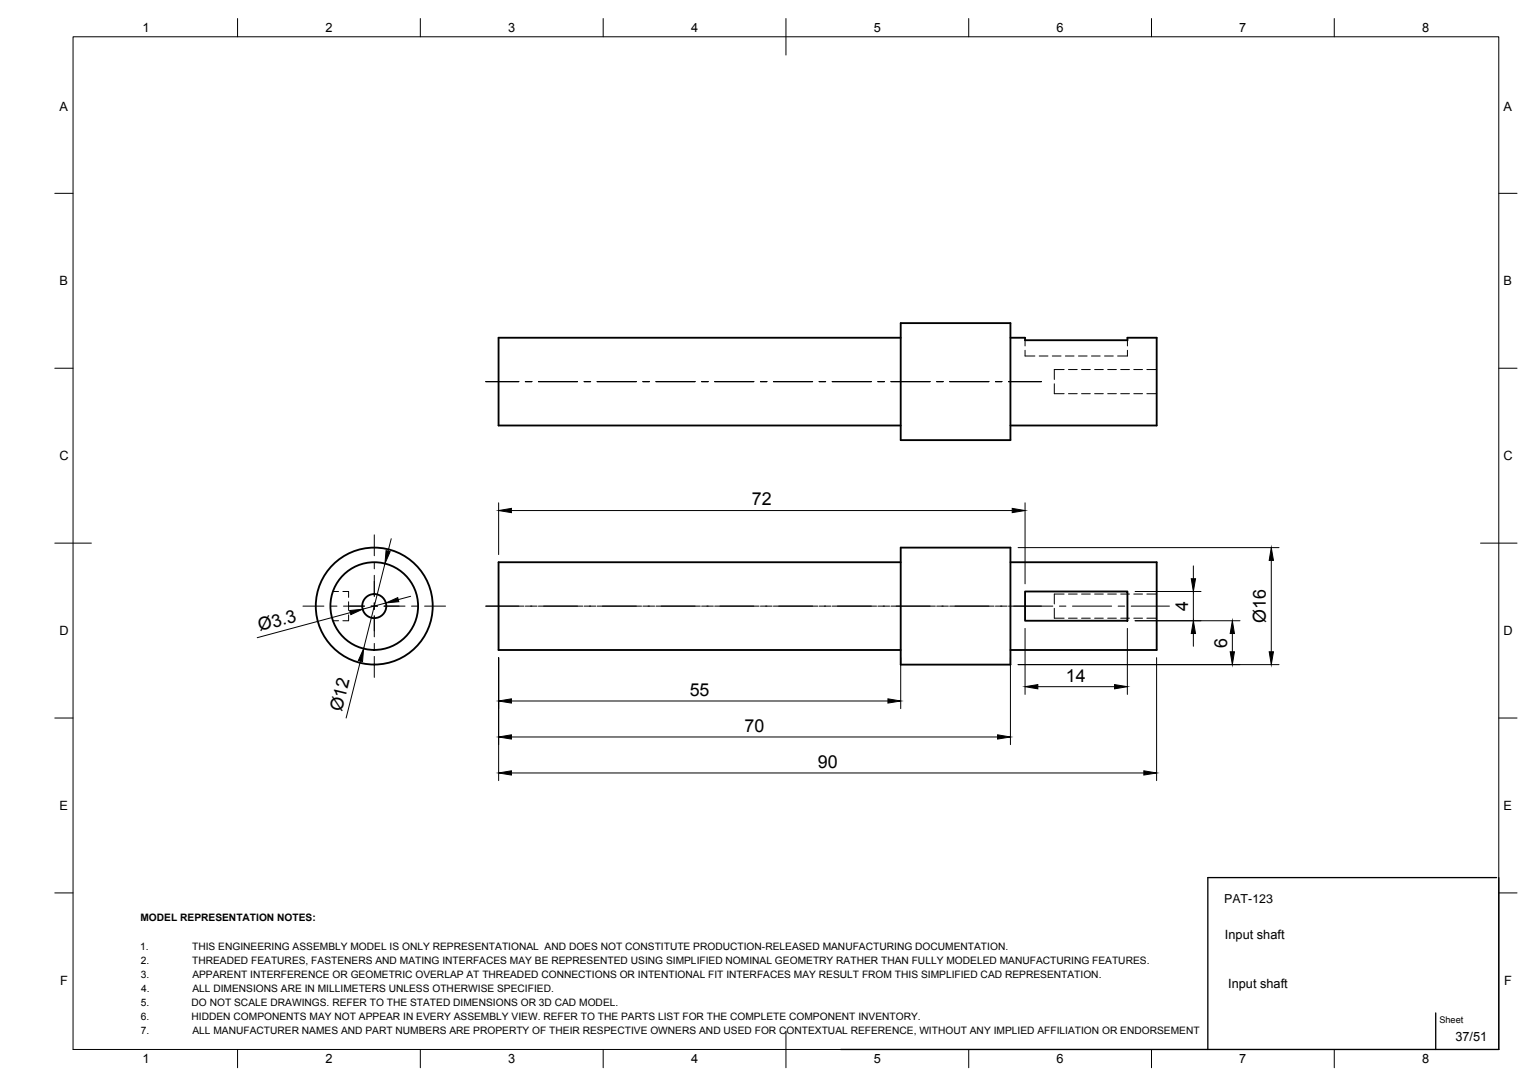
ISO-10303-21;
HEADER;
/* Generated by software containing ST-Developer
 * from STEP Tools, Inc. (www.steptools.com) 
 */

FILE_DESCRIPTION(
/* description */ ('Worm-less right-angle friction wheel drive'),
/* implementation_level */ '2;1');

FILE_NAME(
/* name */ 'Input shaft.step',
/* time_stamp */ '2026-10-28T03:22:36-07:00',
/* author */ (''),
/* organization */ (''),
/* preprocessor_version */ 'ST-DEVELOPER v20.2',
/* originating_system */ 'Autodesk Translation Framework v15.17.0.0',
/* authorisation */ '');

FILE_SCHEMA (('AUTOMOTIVE_DESIGN { 1 0 10303 214 3 1 1 }'));
ENDSEC;

DATA;
#10=MECHANICAL_DESIGN_GEOMETRIC_PRESENTATION_REPRESENTATION('',(#650),#17046);
#549=SHAPE_REPRESENTATION_RELATIONSHIP('SRR','None',#17294,#596);
#596=ADVANCED_BREP_SHAPE_REPRESENTATION('',(#701),#17030);
#650=STYLED_ITEM('',(#17591),#701);
#701=MANIFOLD_SOLID_BREP('Body1',#8208);
#919=FACE_BOUND('',#2229,.T.);
#920=FACE_BOUND('',#2231,.T.);
#921=FACE_BOUND('',#2235,.T.);
#922=FACE_BOUND('',#2237,.T.);
#1125=PLANE('',#9460);
#1126=PLANE('',#9461);
#1127=PLANE('',#9462);
#1128=PLANE('',#9464);
#1129=PLANE('',#9465);
#1130=PLANE('',#9466);
#1131=PLANE('',#9468);
#1132=PLANE('',#9471);
#1133=PLANE('',#9479);
#1134=PLANE('',#9480);
#1551=FACE_OUTER_BOUND('',#2221,.T.);
#1552=FACE_OUTER_BOUND('',#2222,.T.);
#1553=FACE_OUTER_BOUND('',#2223,.T.);
#1554=FACE_OUTER_BOUND('',#2224,.T.);
#1555=FACE_OUTER_BOUND('',#2225,.T.);
#1556=FACE_OUTER_BOUND('',#2226,.T.);
#1557=FACE_OUTER_BOUND('',#2227,.T.);
#1558=FACE_OUTER_BOUND('',#2228,.T.);
#1559=FACE_OUTER_BOUND('',#2230,.T.);
#1560=FACE_OUTER_BOUND('',#2232,.T.);
#1561=FACE_OUTER_BOUND('',#2233,.T.);
#1562=FACE_OUTER_BOUND('',#2234,.T.);
#1563=FACE_OUTER_BOUND('',#2236,.T.);
#1564=FACE_OUTER_BOUND('',#2238,.T.);
#2221=EDGE_LOOP('',(#7038,#7039,#7040,#7041));
#2222=EDGE_LOOP('',(#7042));
#2223=EDGE_LOOP('',(#7043,#7044,#7045,#7046));
#2224=EDGE_LOOP('',(#7047,#7048,#7049,#7050));
#2225=EDGE_LOOP('',(#7051,#7052,#7053,#7054));
#2226=EDGE_LOOP('',(#7055,#7056,#7057,#7058));
#2227=EDGE_LOOP('',(#7059,#7060,#7061,#7062));
#2228=EDGE_LOOP('',(#7063));
#2229=EDGE_LOOP('',(#7064));
#2230=EDGE_LOOP('',(#7065));
#2231=EDGE_LOOP('',(#7066));
#2232=EDGE_LOOP('',(#7067,#7068,#7069,#7070));
#2233=EDGE_LOOP('',(#7071,#7072,#7073,#7074));
#2234=EDGE_LOOP('',(#7075,#7076,#7077,#7078));
#2235=EDGE_LOOP('',(#7079,#7080,#7081,#7082));
#2236=EDGE_LOOP('',(#7083));
#2237=EDGE_LOOP('',(#7084));
#2238=EDGE_LOOP('',(#7085));
#2769=LINE('',#16139,#3309);
#2770=LINE('',#16145,#3310);
#2771=LINE('',#16147,#3311);
#2772=LINE('',#16149,#3312);
#2773=LINE('',#16150,#3313);
#2774=LINE('',#16155,#3314);
#2775=LINE('',#16156,#3315);
#2776=LINE('',#16159,#3316);
#2777=LINE('',#16161,#3317);
#2778=LINE('',#16162,#3318);
#2779=LINE('',#16164,#3319);
#2780=LINE('',#16178,#3320);
#2781=LINE('',#16181,#3321);
#2782=LINE('',#16186,#3322);
#3309=VECTOR('',#11599,0.165);
#3310=VECTOR('',#11606,1.);
#3311=VECTOR('',#11607,1.);
#3312=VECTOR('',#11608,1.);
#3313=VECTOR('',#11609,1.);
#3314=VECTOR('',#11614,1.);
#3315=VECTOR('',#11615,1.);
#3316=VECTOR('',#11618,1.);
#3317=VECTOR('',#11619,1.);
#3318=VECTOR('',#11620,1.);
#3319=VECTOR('',#11623,1.);
#3320=VECTOR('',#11642,0.8);
#3321=VECTOR('',#11645,0.6);
#3322=VECTOR('',#11652,0.6);
#3789=CIRCLE('',#9458,0.165);
#3790=CIRCLE('',#9459,0.165);
#3791=CIRCLE('',#9463,0.6);
#3792=CIRCLE('',#9467,0.6);
#3793=CIRCLE('',#9469,0.8);
#3794=CIRCLE('',#9470,0.6);
#3795=CIRCLE('',#9472,0.8);
#3796=CIRCLE('',#9473,0.6);
#3797=CIRCLE('',#9476,0.6);
#3798=CIRCLE('',#9478,0.6);
#4374=VERTEX_POINT('',#16136);
#4375=VERTEX_POINT('',#16138);
#4376=VERTEX_POINT('',#16143);
#4377=VERTEX_POINT('',#16144);
#4378=VERTEX_POINT('',#16146);
#4379=VERTEX_POINT('',#16148);
#4380=VERTEX_POINT('',#16152);
#4381=VERTEX_POINT('',#16154);
#4382=VERTEX_POINT('',#16158);
#4383=VERTEX_POINT('',#16160);
#4384=VERTEX_POINT('',#16168);
#4385=VERTEX_POINT('',#16170);
#4386=VERTEX_POINT('',#16173);
#4387=VERTEX_POINT('',#16175);
#4388=VERTEX_POINT('',#16180);
#4389=VERTEX_POINT('',#16184);
#5288=EDGE_CURVE('',#4374,#4374,#3789,.T.);
#5289=EDGE_CURVE('',#4374,#4375,#2769,.T.);
#5290=EDGE_CURVE('',#4375,#4375,#3790,.T.);
#5291=EDGE_CURVE('',#4376,#4377,#2770,.T.);
#5292=EDGE_CURVE('',#4376,#4378,#2771,.T.);
#5293=EDGE_CURVE('',#4379,#4378,#2772,.T.);
#5294=EDGE_CURVE('',#4379,#4377,#2773,.T.);
#5295=EDGE_CURVE('',#4377,#4380,#3791,.T.);
#5296=EDGE_CURVE('',#4381,#4379,#2774,.T.);
#5297=EDGE_CURVE('',#4380,#4381,#2775,.T.);
#5298=EDGE_CURVE('',#4380,#4382,#2776,.T.);
#5299=EDGE_CURVE('',#4381,#4383,#2777,.T.);
#5300=EDGE_CURVE('',#4383,#4382,#2778,.T.);
#5301=EDGE_CURVE('',#4378,#4383,#2779,.T.);
#5302=EDGE_CURVE('',#4382,#4376,#3792,.T.);
#5303=EDGE_CURVE('',#4384,#4384,#3793,.T.);
#5304=EDGE_CURVE('',#4385,#4385,#3794,.T.);
#5305=EDGE_CURVE('',#4386,#4386,#3795,.T.);
#5306=EDGE_CURVE('',#4387,#4387,#3796,.T.);
#5307=EDGE_CURVE('',#4384,#4386,#2780,.T.);
#5308=EDGE_CURVE('',#4387,#4388,#2781,.T.);
#5309=EDGE_CURVE('',#4388,#4388,#3797,.T.);
#5310=EDGE_CURVE('',#4389,#4389,#3798,.T.);
#5311=EDGE_CURVE('',#4389,#4385,#2782,.T.);
#7038=ORIENTED_EDGE('',*,*,#5288,.F.);
#7039=ORIENTED_EDGE('',*,*,#5289,.T.);
#7040=ORIENTED_EDGE('',*,*,#5290,.F.);
#7041=ORIENTED_EDGE('',*,*,#5289,.F.);
#7042=ORIENTED_EDGE('',*,*,#5288,.T.);
#7043=ORIENTED_EDGE('',*,*,#5291,.F.);
#7044=ORIENTED_EDGE('',*,*,#5292,.T.);
#7045=ORIENTED_EDGE('',*,*,#5293,.F.);
#7046=ORIENTED_EDGE('',*,*,#5294,.T.);
#7047=ORIENTED_EDGE('',*,*,#5295,.F.);
#7048=ORIENTED_EDGE('',*,*,#5294,.F.);
#7049=ORIENTED_EDGE('',*,*,#5296,.F.);
#7050=ORIENTED_EDGE('',*,*,#5297,.F.);
#7051=ORIENTED_EDGE('',*,*,#5298,.F.);
#7052=ORIENTED_EDGE('',*,*,#5297,.T.);
#7053=ORIENTED_EDGE('',*,*,#5299,.T.);
#7054=ORIENTED_EDGE('',*,*,#5300,.T.);
#7055=ORIENTED_EDGE('',*,*,#5296,.T.);
#7056=ORIENTED_EDGE('',*,*,#5293,.T.);
#7057=ORIENTED_EDGE('',*,*,#5301,.T.);
#7058=ORIENTED_EDGE('',*,*,#5299,.F.);
#7059=ORIENTED_EDGE('',*,*,#5302,.F.);
#7060=ORIENTED_EDGE('',*,*,#5300,.F.);
#7061=ORIENTED_EDGE('',*,*,#5301,.F.);
#7062=ORIENTED_EDGE('',*,*,#5292,.F.);
#7063=ORIENTED_EDGE('',*,*,#5303,.T.);
#7064=ORIENTED_EDGE('',*,*,#5304,.F.);
#7065=ORIENTED_EDGE('',*,*,#5305,.F.);
#7066=ORIENTED_EDGE('',*,*,#5306,.F.);
#7067=ORIENTED_EDGE('',*,*,#5303,.F.);
#7068=ORIENTED_EDGE('',*,*,#5307,.T.);
#7069=ORIENTED_EDGE('',*,*,#5305,.T.);
#7070=ORIENTED_EDGE('',*,*,#5307,.F.);
#7071=ORIENTED_EDGE('',*,*,#5306,.T.);
#7072=ORIENTED_EDGE('',*,*,#5308,.T.);
#7073=ORIENTED_EDGE('',*,*,#5309,.T.);
#7074=ORIENTED_EDGE('',*,*,#5308,.F.);
#7075=ORIENTED_EDGE('',*,*,#5310,.F.);
#7076=ORIENTED_EDGE('',*,*,#5311,.T.);
#7077=ORIENTED_EDGE('',*,*,#5304,.T.);
#7078=ORIENTED_EDGE('',*,*,#5311,.F.);
#7079=ORIENTED_EDGE('',*,*,#5298,.T.);
#7080=ORIENTED_EDGE('',*,*,#5302,.T.);
#7081=ORIENTED_EDGE('',*,*,#5291,.T.);
#7082=ORIENTED_EDGE('',*,*,#5295,.T.);
#7083=ORIENTED_EDGE('',*,*,#5310,.T.);
#7084=ORIENTED_EDGE('',*,*,#5290,.T.);
#7085=ORIENTED_EDGE('',*,*,#5309,.F.);
#7665=CYLINDRICAL_SURFACE('',#9457,0.165);
#7666=CYLINDRICAL_SURFACE('',#9474,0.8);
#7667=CYLINDRICAL_SURFACE('',#9475,0.6);
#7668=CYLINDRICAL_SURFACE('',#9477,0.6);
#8043=ADVANCED_FACE('',(#1551),#7665,.F.);
#8044=ADVANCED_FACE('',(#1552),#1125,.T.);
#8045=ADVANCED_FACE('',(#1553),#1126,.F.);
#8046=ADVANCED_FACE('',(#1554),#1127,.T.);
#8047=ADVANCED_FACE('',(#1555),#1128,.F.);
#8048=ADVANCED_FACE('',(#1556),#1129,.F.);
#8049=ADVANCED_FACE('',(#1557),#1130,.F.);
#8050=ADVANCED_FACE('',(#1558,#919),#1131,.T.);
#8051=ADVANCED_FACE('',(#1559,#920),#1132,.F.);
#8052=ADVANCED_FACE('',(#1560),#7666,.T.);
#8053=ADVANCED_FACE('',(#1561),#7667,.T.);
#8054=ADVANCED_FACE('',(#1562,#921),#7668,.T.);
#8055=ADVANCED_FACE('',(#1563,#922),#1133,.T.);
#8056=ADVANCED_FACE('',(#1564),#1134,.F.);
#8208=CLOSED_SHELL('',(#8043,#8044,#8045,#8046,#8047,#8048,#8049,#8050,
#8051,#8052,#8053,#8054,#8055,#8056));
#9456=AXIS2_PLACEMENT_3D('',#16134,#11593,#11594);
#9457=AXIS2_PLACEMENT_3D('',#16135,#11595,#11596);
#9458=AXIS2_PLACEMENT_3D('',#16137,#11597,#11598);
#9459=AXIS2_PLACEMENT_3D('',#16140,#11600,#11601);
#9460=AXIS2_PLACEMENT_3D('',#16141,#11602,#11603);
#9461=AXIS2_PLACEMENT_3D('',#16142,#11604,#11605);
#9462=AXIS2_PLACEMENT_3D('',#16151,#11610,#11611);
#9463=AXIS2_PLACEMENT_3D('',#16153,#11612,#11613);
#9464=AXIS2_PLACEMENT_3D('',#16157,#11616,#11617);
#9465=AXIS2_PLACEMENT_3D('',#16163,#11621,#11622);
#9466=AXIS2_PLACEMENT_3D('',#16165,#11624,#11625);
#9467=AXIS2_PLACEMENT_3D('',#16166,#11626,#11627);
#9468=AXIS2_PLACEMENT_3D('',#16167,#11628,#11629);
#9469=AXIS2_PLACEMENT_3D('',#16169,#11630,#11631);
#9470=AXIS2_PLACEMENT_3D('',#16171,#11632,#11633);
#9471=AXIS2_PLACEMENT_3D('',#16172,#11634,#11635);
#9472=AXIS2_PLACEMENT_3D('',#16174,#11636,#11637);
#9473=AXIS2_PLACEMENT_3D('',#16176,#11638,#11639);
#9474=AXIS2_PLACEMENT_3D('',#16177,#11640,#11641);
#9475=AXIS2_PLACEMENT_3D('',#16179,#11643,#11644);
#9476=AXIS2_PLACEMENT_3D('',#16182,#11646,#11647);
#9477=AXIS2_PLACEMENT_3D('',#16183,#11648,#11649);
#9478=AXIS2_PLACEMENT_3D('',#16185,#11650,#11651);
#9479=AXIS2_PLACEMENT_3D('',#16187,#11653,#11654);
#9480=AXIS2_PLACEMENT_3D('',#16188,#11655,#11656);
#11593=DIRECTION('axis',(0.,0.,1.));
#11594=DIRECTION('refdir',(1.,0.,0.));
#11595=DIRECTION('center_axis',(0.,1.,0.));
#11596=DIRECTION('ref_axis',(1.,0.,0.));
#11597=DIRECTION('center_axis',(0.,1.,0.));
#11598=DIRECTION('ref_axis',(1.,0.,0.));
#11599=DIRECTION('',(0.,1.,0.));
#11600=DIRECTION('center_axis',(0.,-1.,0.));
#11601=DIRECTION('ref_axis',(1.,0.,0.));
#11602=DIRECTION('center_axis',(0.,1.,0.));
#11603=DIRECTION('ref_axis',(1.,0.,0.));
#11604=DIRECTION('center_axis',(-1.,0.,0.));
#11605=DIRECTION('ref_axis',(0.,0.,1.));
#11606=DIRECTION('',(0.,-1.,0.));
#11607=DIRECTION('',(0.,0.,1.));
#11608=DIRECTION('',(0.,1.,0.));
#11609=DIRECTION('',(0.,0.,-1.));
#11610=DIRECTION('center_axis',(0.,1.,0.));
#11611=DIRECTION('ref_axis',(1.,0.,0.));
#11612=DIRECTION('center_axis',(0.,-1.,0.));
#11613=DIRECTION('ref_axis',(1.,0.,0.));
#11614=DIRECTION('',(-1.,0.,0.));
#11615=DIRECTION('',(0.,0.,1.));
#11616=DIRECTION('center_axis',(1.,0.,0.));
#11617=DIRECTION('ref_axis',(0.,0.,-1.));
#11618=DIRECTION('',(0.,1.,0.));
#11619=DIRECTION('',(0.,1.,0.));
#11620=DIRECTION('',(0.,0.,-1.));
#11621=DIRECTION('center_axis',(0.,0.,1.));
#11622=DIRECTION('ref_axis',(1.,0.,0.));
#11623=DIRECTION('',(1.,0.,0.));
#11624=DIRECTION('center_axis',(0.,1.,0.));
#11625=DIRECTION('ref_axis',(0.,0.,1.));
#11626=DIRECTION('center_axis',(0.,1.,0.));
#11627=DIRECTION('ref_axis',(1.,0.,0.));
#11628=DIRECTION('center_axis',(0.,1.,0.));
#11629=DIRECTION('ref_axis',(1.,0.,0.));
#11630=DIRECTION('center_axis',(0.,1.,0.));
#11631=DIRECTION('ref_axis',(1.,0.,0.));
#11632=DIRECTION('center_axis',(0.,1.,0.));
#11633=DIRECTION('ref_axis',(1.,0.,0.));
#11634=DIRECTION('center_axis',(0.,1.,0.));
#11635=DIRECTION('ref_axis',(1.,0.,0.));
#11636=DIRECTION('center_axis',(0.,1.,0.));
#11637=DIRECTION('ref_axis',(1.,0.,0.));
#11638=DIRECTION('center_axis',(0.,-1.,0.));
#11639=DIRECTION('ref_axis',(1.,0.,0.));
#11640=DIRECTION('center_axis',(0.,1.,0.));
#11641=DIRECTION('ref_axis',(1.,0.,0.));
#11642=DIRECTION('',(0.,-1.,0.));
#11643=DIRECTION('center_axis',(0.,1.,0.));
#11644=DIRECTION('ref_axis',(1.,0.,0.));
#11645=DIRECTION('',(0.,-1.,0.));
#11646=DIRECTION('center_axis',(0.,1.,0.));
#11647=DIRECTION('ref_axis',(1.,0.,0.));
#11648=DIRECTION('center_axis',(0.,1.,0.));
#11649=DIRECTION('ref_axis',(1.,0.,0.));
#11650=DIRECTION('center_axis',(0.,1.,0.));
#11651=DIRECTION('ref_axis',(1.,0.,0.));
#11652=DIRECTION('',(0.,-1.,0.));
#11653=DIRECTION('center_axis',(0.,1.,0.));
#11654=DIRECTION('ref_axis',(1.,0.,0.));
#11655=DIRECTION('center_axis',(0.,1.,0.));
#11656=DIRECTION('ref_axis',(1.,0.,0.));
#16134=CARTESIAN_POINT('',(0.,0.,0.));
#16135=CARTESIAN_POINT('Origin',(0.,-1.4,7.));
#16136=CARTESIAN_POINT('',(-0.165,-1.4,7.));
#16137=CARTESIAN_POINT('Origin',(0.,-1.4,7.));
#16138=CARTESIAN_POINT('',(-0.165,0.,7.));
#16139=CARTESIAN_POINT('',(-0.165,-1.4,7.));
#16140=CARTESIAN_POINT('Origin',(0.,0.,7.));
#16141=CARTESIAN_POINT('Origin',(0.,-1.4,7.));
#16142=CARTESIAN_POINT('Origin',(-0.2,-1.8,6.3));
#16143=CARTESIAN_POINT('',(-0.2,-0.4,6.43431457505076));
#16144=CARTESIAN_POINT('',(-0.2,-1.8,6.43431457505076));
#16145=CARTESIAN_POINT('',(-0.2,-9.,6.43431457505076));
#16146=CARTESIAN_POINT('',(-0.2,-0.4,6.65));
#16147=CARTESIAN_POINT('',(-0.2,-0.4,6.65));
#16148=CARTESIAN_POINT('',(-0.2,-1.8,6.65));
#16149=CARTESIAN_POINT('',(-0.2,-1.8,6.65));
#16150=CARTESIAN_POINT('',(-0.2,-1.8,6.65));
#16151=CARTESIAN_POINT('Origin',(0.,-1.8,6.475));
#16152=CARTESIAN_POINT('',(0.2,-1.8,6.43431457505076));
#16153=CARTESIAN_POINT('Origin',(0.,-1.8,7.));
#16154=CARTESIAN_POINT('',(0.2,-1.8,6.65));
#16155=CARTESIAN_POINT('',(0.2,-1.8,6.65));
#16156=CARTESIAN_POINT('',(0.2,-1.8,6.3));
#16157=CARTESIAN_POINT('Origin',(0.2,-1.8,6.65));
#16158=CARTESIAN_POINT('',(0.2,-0.4,6.43431457505076));
#16159=CARTESIAN_POINT('',(0.2,-9.,6.43431457505076));
#16160=CARTESIAN_POINT('',(0.2,-0.4,6.65));
#16161=CARTESIAN_POINT('',(0.2,-1.8,6.65));
#16162=CARTESIAN_POINT('',(0.2,-0.4,6.3));
#16163=CARTESIAN_POINT('Origin',(-0.2,-1.8,6.65));
#16164=CARTESIAN_POINT('',(0.2,-0.4,6.65));
#16165=CARTESIAN_POINT('Origin',(0.,-0.4,6.475));
#16166=CARTESIAN_POINT('Origin',(0.,-0.4,7.));
#16167=CARTESIAN_POINT('Origin',(0.,-2.,7.));
#16168=CARTESIAN_POINT('',(-0.8,-2.,7.));
#16169=CARTESIAN_POINT('Origin',(0.,-2.,7.));
#16170=CARTESIAN_POINT('',(-0.6,-2.,7.));
#16171=CARTESIAN_POINT('Origin',(0.,-2.,7.));
#16172=CARTESIAN_POINT('Origin',(0.,-3.5,7.));
#16173=CARTESIAN_POINT('',(-0.8,-3.5,7.));
#16174=CARTESIAN_POINT('Origin',(0.,-3.5,7.));
#16175=CARTESIAN_POINT('',(-0.6,-3.5,7.));
#16176=CARTESIAN_POINT('Origin',(0.,-3.5,7.));
#16177=CARTESIAN_POINT('Origin',(0.,-3.5,7.));
#16178=CARTESIAN_POINT('',(-0.8,-3.5,7.));
#16179=CARTESIAN_POINT('Origin',(0.,-9.,7.));
#16180=CARTESIAN_POINT('',(-0.6,-9.,7.));
#16181=CARTESIAN_POINT('',(-0.6,-9.,7.));
#16182=CARTESIAN_POINT('Origin',(0.,-9.,7.));
#16183=CARTESIAN_POINT('Origin',(0.,-9.,7.));
#16184=CARTESIAN_POINT('',(-0.6,0.,7.));
#16185=CARTESIAN_POINT('Origin',(0.,0.,7.));
#16186=CARTESIAN_POINT('',(-0.6,-9.,7.));
#16187=CARTESIAN_POINT('Origin',(0.,0.,7.));
#16188=CARTESIAN_POINT('Origin',(0.,-9.,7.));
#16977=UNCERTAINTY_MEASURE_WITH_UNIT(LENGTH_MEASURE(0.001),#17047,
'DISTANCE_ACCURACY_VALUE',
'Maximum model space distance between geometric entities at asserted c
onnectivities');
#16993=UNCERTAINTY_MEASURE_WITH_UNIT(LENGTH_MEASURE(0.001),#17047,
'DISTANCE_ACCURACY_VALUE',
'Maximum model space distance between geometric entities at asserted c
onnectivities');
#17030=(
GEOMETRIC_REPRESENTATION_CONTEXT(3)
GLOBAL_UNCERTAINTY_ASSIGNED_CONTEXT((#16977))
GLOBAL_UNIT_ASSIGNED_CONTEXT((#17047,#17049,#17050))
REPRESENTATION_CONTEXT('','3D')
);
#17046=(
GEOMETRIC_REPRESENTATION_CONTEXT(3)
GLOBAL_UNCERTAINTY_ASSIGNED_CONTEXT((#16993))
GLOBAL_UNIT_ASSIGNED_CONTEXT((#17047,#17049,#17050))
REPRESENTATION_CONTEXT('','3D')
);
#17047=(
LENGTH_UNIT()
NAMED_UNIT(*)
SI_UNIT(.CENTI.,.METRE.)
);
#17049=(
NAMED_UNIT(*)
PLANE_ANGLE_UNIT()
SI_UNIT($,.RADIAN.)
);
#17050=(
NAMED_UNIT(*)
SI_UNIT($,.STERADIAN.)
SOLID_ANGLE_UNIT()
);
#17087=SHAPE_DEFINITION_REPRESENTATION(#17144,#17294);
#17144=PRODUCT_DEFINITION_SHAPE('',$,#17347);
#17294=SHAPE_REPRESENTATION('',(#9456),#17030);
#17310=PRODUCT_DEFINITION_CONTEXT('part definition',#17468,'design');
#17347=PRODUCT_DEFINITION('Input shaft','Input shaft',#17399,#17310);
#17399=PRODUCT_DEFINITION_FORMATION('',$,#17506);
#17468=APPLICATION_CONTEXT(
'Core Data for Automotive Mechanical Design Process');
#17469=PRODUCT_CONTEXT('part definition',#17468,'mechanical');
#17506=PRODUCT('Input shaft','Input shaft','Input shaft',(#17469));
#17585=COLOUR_RGB('Grey',0.48,0.52,0.57);
#17586=FILL_AREA_STYLE_COLOUR('',#17585);
#17587=FILL_AREA_STYLE('',(#17586));
#17588=SURFACE_STYLE_FILL_AREA(#17587);
#17589=SURFACE_SIDE_STYLE('',(#17588));
#17590=SURFACE_STYLE_USAGE(.BOTH.,#17589);
#17591=PRESENTATION_STYLE_ASSIGNMENT((#17590));
ENDSEC;
END-ISO-10303-21;
